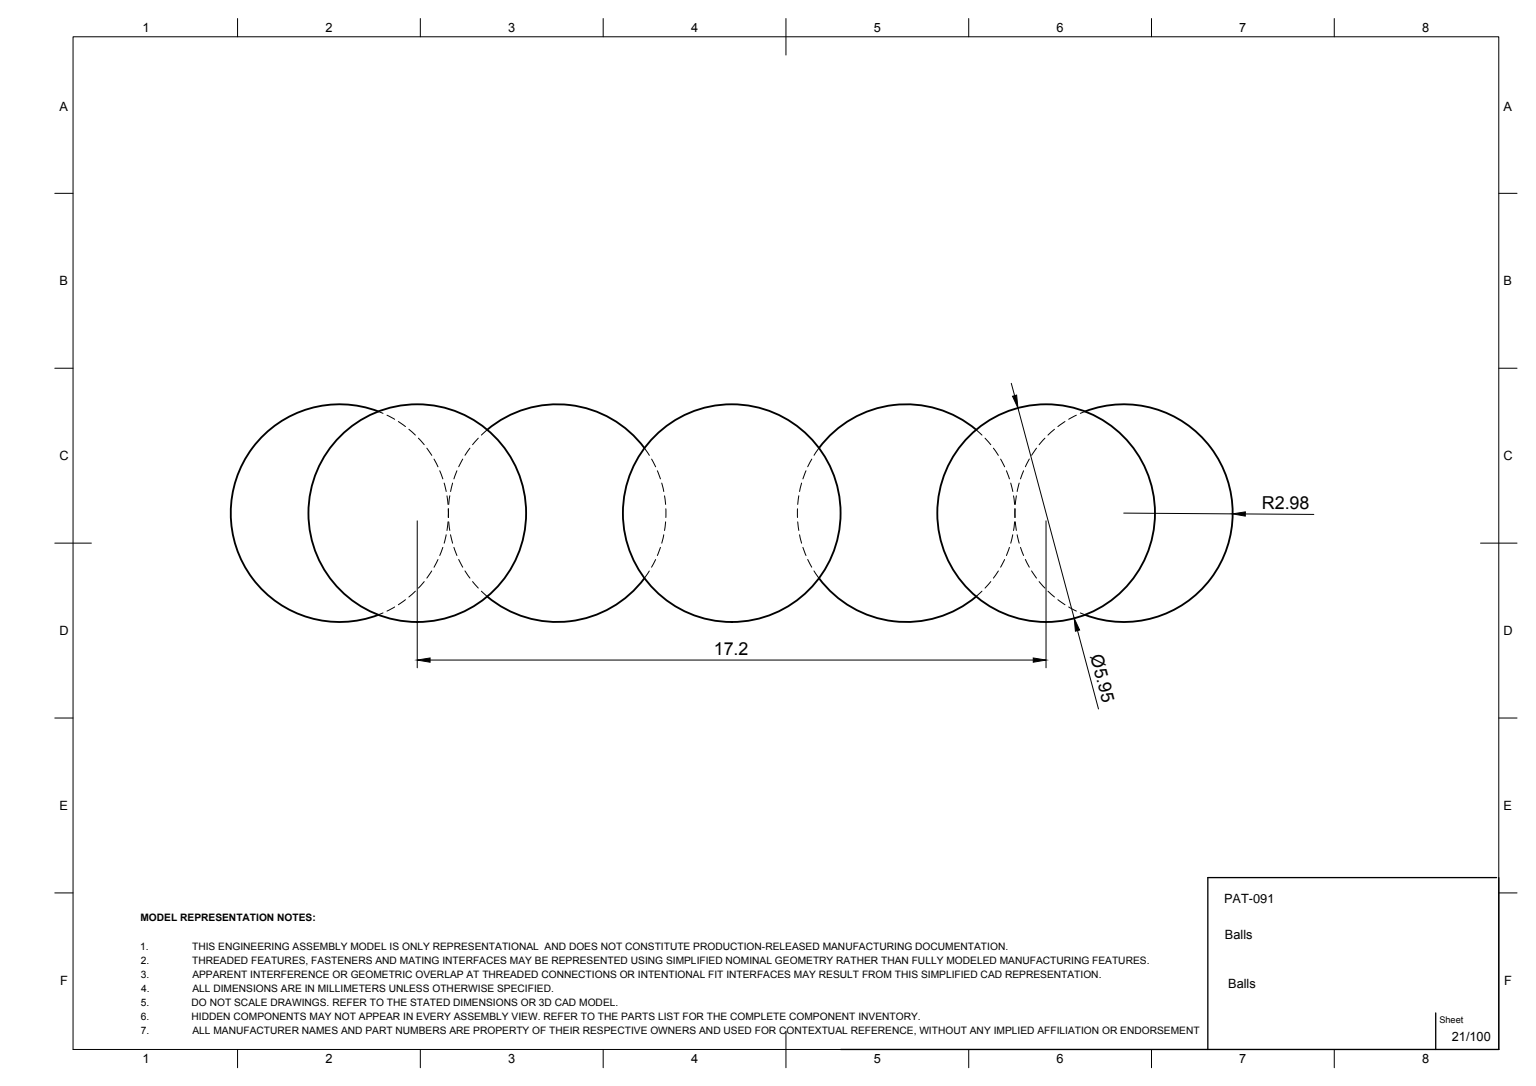
ISO-10303-21;
HEADER;
/* Generated by software containing ST-Developer
 * from STEP Tools, Inc. (www.steptools.com) 
 */

FILE_DESCRIPTION(
/* description */ ('PAT-091'),
/* implementation_level */ '2;1');

FILE_NAME(
/* name */ 'Balls.step',
/* time_stamp */ '2026-10-27T15:34:44-07:00',
/* author */ (''),
/* organization */ (''),
/* preprocessor_version */ 'ST-DEVELOPER v20.2',
/* originating_system */ 'Autodesk Translation Framework v15.17.0.0',
/* authorisation */ '');

FILE_SCHEMA (('AUTOMOTIVE_DESIGN { 1 0 10303 214 3 1 1 }'));
ENDSEC;

DATA;
#10=MECHANICAL_DESIGN_GEOMETRIC_PRESENTATION_REPRESENTATION('',(#1072,#1073,#1074,#1075,#1076,#1077,#1078),#25100);
#14=SPHERICAL_SURFACE('',#16174,0.29765);
#15=SPHERICAL_SURFACE('',#16176,0.29765);
#16=SPHERICAL_SURFACE('',#16178,0.29765);
#17=SPHERICAL_SURFACE('',#16180,0.29765);
#18=SPHERICAL_SURFACE('',#16182,0.29765);
#19=SPHERICAL_SURFACE('',#16184,0.29765);
#20=SPHERICAL_SURFACE('',#16186,0.29765);
#852=SHAPE_REPRESENTATION_RELATIONSHIP('SRR','None',#25620,#962);
#962=ADVANCED_BREP_SHAPE_REPRESENTATION('',(#1193,#1194,#1195,#1196,#1197,
#1198,#1199),#25090);
#1072=STYLED_ITEM('',(#26191),#1193);
#1073=STYLED_ITEM('',(#26191),#1194);
#1074=STYLED_ITEM('',(#26191),#1195);
#1075=STYLED_ITEM('',(#26191),#1196);
#1076=STYLED_ITEM('',(#26191),#1197);
#1077=STYLED_ITEM('',(#26191),#1198);
#1078=STYLED_ITEM('',(#26191),#1199);
#1193=MANIFOLD_SOLID_BREP('Body1',#13352);
#1194=MANIFOLD_SOLID_BREP('Body2',#13353);
#1195=MANIFOLD_SOLID_BREP('Body3',#13354);
#1196=MANIFOLD_SOLID_BREP('Body4',#13355);
#1197=MANIFOLD_SOLID_BREP('Body5',#13356);
#1198=MANIFOLD_SOLID_BREP('Body6',#13357);
#1199=MANIFOLD_SOLID_BREP('Body7',#13358);
#2791=FACE_OUTER_BOUND('',#4015,.T.);
#2792=FACE_OUTER_BOUND('',#4016,.T.);
#2793=FACE_OUTER_BOUND('',#4017,.T.);
#2794=FACE_OUTER_BOUND('',#4018,.T.);
#2795=FACE_OUTER_BOUND('',#4019,.T.);
#2796=FACE_OUTER_BOUND('',#4020,.T.);
#2797=FACE_OUTER_BOUND('',#4021,.T.);
#4015=EDGE_LOOP('',(#11772,#11773));
#4016=EDGE_LOOP('',(#11774,#11775));
#4017=EDGE_LOOP('',(#11776,#11777));
#4018=EDGE_LOOP('',(#11778,#11779));
#4019=EDGE_LOOP('',(#11780,#11781));
#4020=EDGE_LOOP('',(#11782,#11783));
#4021=EDGE_LOOP('',(#11784,#11785));
#6280=CIRCLE('',#16175,0.29765);
#6281=CIRCLE('',#16177,0.29765);
#6282=CIRCLE('',#16179,0.29765);
#6283=CIRCLE('',#16181,0.29765);
#6284=CIRCLE('',#16183,0.29765);
#6285=CIRCLE('',#16185,0.29765);
#6286=CIRCLE('',#16187,0.29765);
#7311=VERTEX_POINT('',#24268);
#7312=VERTEX_POINT('',#24269);
#7313=VERTEX_POINT('',#24272);
#7314=VERTEX_POINT('',#24273);
#7315=VERTEX_POINT('',#24276);
#7316=VERTEX_POINT('',#24277);
#7317=VERTEX_POINT('',#24280);
#7318=VERTEX_POINT('',#24281);
#7319=VERTEX_POINT('',#24284);
#7320=VERTEX_POINT('',#24285);
#7321=VERTEX_POINT('',#24288);
#7322=VERTEX_POINT('',#24289);
#7323=VERTEX_POINT('',#24292);
#7324=VERTEX_POINT('',#24293);
#8821=EDGE_CURVE('',#7311,#7312,#6280,.T.);
#8822=EDGE_CURVE('',#7313,#7314,#6281,.T.);
#8823=EDGE_CURVE('',#7315,#7316,#6282,.T.);
#8824=EDGE_CURVE('',#7317,#7318,#6283,.T.);
#8825=EDGE_CURVE('',#7319,#7320,#6284,.T.);
#8826=EDGE_CURVE('',#7321,#7322,#6285,.T.);
#8827=EDGE_CURVE('',#7323,#7324,#6286,.T.);
#11772=ORIENTED_EDGE('',*,*,#8821,.T.);
#11773=ORIENTED_EDGE('',*,*,#8821,.F.);
#11774=ORIENTED_EDGE('',*,*,#8822,.T.);
#11775=ORIENTED_EDGE('',*,*,#8822,.F.);
#11776=ORIENTED_EDGE('',*,*,#8823,.T.);
#11777=ORIENTED_EDGE('',*,*,#8823,.F.);
#11778=ORIENTED_EDGE('',*,*,#8824,.T.);
#11779=ORIENTED_EDGE('',*,*,#8824,.F.);
#11780=ORIENTED_EDGE('',*,*,#8825,.T.);
#11781=ORIENTED_EDGE('',*,*,#8825,.F.);
#11782=ORIENTED_EDGE('',*,*,#8826,.T.);
#11783=ORIENTED_EDGE('',*,*,#8826,.F.);
#11784=ORIENTED_EDGE('',*,*,#8827,.T.);
#11785=ORIENTED_EDGE('',*,*,#8827,.F.);
#13158=ADVANCED_FACE('',(#2791),#14,.T.);
#13159=ADVANCED_FACE('',(#2792),#15,.T.);
#13160=ADVANCED_FACE('',(#2793),#16,.T.);
#13161=ADVANCED_FACE('',(#2794),#17,.T.);
#13162=ADVANCED_FACE('',(#2795),#18,.T.);
#13163=ADVANCED_FACE('',(#2796),#19,.T.);
#13164=ADVANCED_FACE('',(#2797),#20,.T.);
#13352=CLOSED_SHELL('',(#13158));
#13353=CLOSED_SHELL('',(#13159));
#13354=CLOSED_SHELL('',(#13160));
#13355=CLOSED_SHELL('',(#13161));
#13356=CLOSED_SHELL('',(#13162));
#13357=CLOSED_SHELL('',(#13163));
#13358=CLOSED_SHELL('',(#13164));
#16173=AXIS2_PLACEMENT_3D('',#24266,#20364,#20365);
#16174=AXIS2_PLACEMENT_3D('',#24267,#20366,#20367);
#16175=AXIS2_PLACEMENT_3D('',#24270,#20368,#20369);
#16176=AXIS2_PLACEMENT_3D('',#24271,#20370,#20371);
#16177=AXIS2_PLACEMENT_3D('',#24274,#20372,#20373);
#16178=AXIS2_PLACEMENT_3D('',#24275,#20374,#20375);
#16179=AXIS2_PLACEMENT_3D('',#24278,#20376,#20377);
#16180=AXIS2_PLACEMENT_3D('',#24279,#20378,#20379);
#16181=AXIS2_PLACEMENT_3D('',#24282,#20380,#20381);
#16182=AXIS2_PLACEMENT_3D('',#24283,#20382,#20383);
#16183=AXIS2_PLACEMENT_3D('',#24286,#20384,#20385);
#16184=AXIS2_PLACEMENT_3D('',#24287,#20386,#20387);
#16185=AXIS2_PLACEMENT_3D('',#24290,#20388,#20389);
#16186=AXIS2_PLACEMENT_3D('',#24291,#20390,#20391);
#16187=AXIS2_PLACEMENT_3D('',#24294,#20392,#20393);
#20364=DIRECTION('axis',(0.,0.,1.));
#20365=DIRECTION('refdir',(1.,0.,0.));
#20366=DIRECTION('center_axis',(0.,0.,1.));
#20367=DIRECTION('ref_axis',(1.,0.,0.));
#20368=DIRECTION('center_axis',(1.22464679914735E-16,-1.,0.));
#20369=DIRECTION('ref_axis',(-1.,-1.22464679914735E-16,0.));
#20370=DIRECTION('center_axis',(0.78183148246803,0.,0.623489801858733));
#20371=DIRECTION('ref_axis',(0.623489801858734,0.,-0.78183148246803));
#20372=DIRECTION('center_axis',(7.63554790147315E-17,-1.,-9.57467422477103E-17));
#20373=DIRECTION('ref_axis',(-0.623489801858734,-1.22464679914735E-16,0.78183148246803));
#20374=DIRECTION('center_axis',(0.974927912181824,0.,-0.222520933956314));
#20375=DIRECTION('ref_axis',(-0.222520933956314,0.,-0.974927912181824));
#20376=DIRECTION('center_axis',(-2.7250954951288E-17,-1.,-1.19394234705288E-16));
#20377=DIRECTION('ref_axis',(0.222520933956314,-1.22464679914735E-16,0.974927912181824));
#20378=DIRECTION('center_axis',(0.433883739117558,0.,-0.900968867902419));
#20379=DIRECTION('ref_axis',(-0.900968867902419,0.,-0.433883739117558));
#20380=DIRECTION('center_axis',(-1.10336864020811E-16,-1.,-5.31354332312403E-17));
#20381=DIRECTION('ref_axis',(0.900968867902419,-1.22464679914735E-16,0.433883739117558));
#20382=DIRECTION('center_axis',(-0.433883739117558,0.,-0.900968867902419));
#20383=DIRECTION('ref_axis',(-0.900968867902419,0.,0.433883739117558));
#20384=DIRECTION('center_axis',(-1.10336864020811E-16,-1.,5.31354332312403E-17));
#20385=DIRECTION('ref_axis',(0.900968867902419,-1.22464679914735E-16,-0.433883739117558));
#20386=DIRECTION('center_axis',(-0.974927912181824,0.,-0.222520933956314));
#20387=DIRECTION('ref_axis',(-0.222520933956315,0.,0.974927912181824));
#20388=DIRECTION('center_axis',(-2.7250954951288E-17,-1.,1.19394234705288E-16));
#20389=DIRECTION('ref_axis',(0.222520933956315,-1.22464679914735E-16,-0.974927912181824));
#20390=DIRECTION('center_axis',(-0.78183148246803,0.,0.623489801858734));
#20391=DIRECTION('ref_axis',(0.623489801858733,0.,0.78183148246803));
#20392=DIRECTION('center_axis',(7.63554790147315E-17,-1.,9.57467422477103E-17));
#20393=DIRECTION('ref_axis',(-0.623489801858733,-1.22464679914735E-16,-0.78183148246803));
#24266=CARTESIAN_POINT('',(0.,0.,0.));
#24267=CARTESIAN_POINT('Origin',(1.1,0.,0.));
#24268=CARTESIAN_POINT('',(1.1,-2.23201749654651E-33,0.29765));
#24269=CARTESIAN_POINT('',(1.1,-2.23201749654651E-33,-0.29765));
#24270=CARTESIAN_POINT('Origin',(1.1,0.,0.));
#24271=CARTESIAN_POINT('Origin',(0.685838782044607,0.,-0.860014630714833));
#24272=CARTESIAN_POINT('',(0.918550922801216,-5.31350540756609E-33,-0.674432891191581));
#24273=CARTESIAN_POINT('',(0.453126641287998,8.49470414473068E-34,-1.04559637023808));
#24274=CARTESIAN_POINT('Origin',(0.685838782044607,0.,-0.860014630714833));
#24275=CARTESIAN_POINT('Origin',(-0.244773027351946,0.,-1.07242070340001));
#24276=CARTESIAN_POINT('',(0.0454142657089739,-2.23201749654651E-33,-1.1386540593921));
#24277=CARTESIAN_POINT('',(-0.534960320412865,-2.23201749654651E-33,-1.00618734740791));
#24278=CARTESIAN_POINT('Origin',(-0.244773027351946,0.,-1.07242070340001));
#24279=CARTESIAN_POINT('Origin',(-0.991065754692661,0.,-0.477272113029314));
#24280=CARTESIAN_POINT('',(-0.86192025974432,8.49470414473067E-34,-0.745445496560469));
#24281=CARTESIAN_POINT('',(-1.120211249641,-5.31350540756609E-33,-0.209098729498159));
#24282=CARTESIAN_POINT('Origin',(-0.991065754692661,0.,-0.477272113029314));
#24283=CARTESIAN_POINT('Origin',(-0.991065754692661,0.,0.477272113029314));
#24284=CARTESIAN_POINT('',(-1.120211249641,-2.23201749654651E-33,0.209098729498159));
#24285=CARTESIAN_POINT('',(-0.86192025974432,-2.23201749654651E-33,0.745445496560469));
#24286=CARTESIAN_POINT('Origin',(-0.991065754692661,0.,0.477272113029314));
#24287=CARTESIAN_POINT('Origin',(-0.244773027351946,0.,1.07242070340001));
#24288=CARTESIAN_POINT('',(-0.534960320412866,-2.23201749654651E-33,1.00618734740791));
#24289=CARTESIAN_POINT('',(0.0454142657089737,-2.23201749654651E-33,1.1386540593921));
#24290=CARTESIAN_POINT('Origin',(-0.244773027351946,0.,1.07242070340001));
#24291=CARTESIAN_POINT('Origin',(0.685838782044607,0.,0.860014630714833));
#24292=CARTESIAN_POINT('',(0.453126641287998,-2.23201749654651E-33,1.04559637023808));
#24293=CARTESIAN_POINT('',(0.918550922801216,-2.23201749654651E-33,0.674432891191581));
#24294=CARTESIAN_POINT('Origin',(0.685838782044607,0.,0.860014630714833));
#24969=UNCERTAINTY_MEASURE_WITH_UNIT(LENGTH_MEASURE(0.001),#25101,
'DISTANCE_ACCURACY_VALUE',
'Maximum model space distance between geometric entities at asserted c
onnectivities');
#24979=UNCERTAINTY_MEASURE_WITH_UNIT(LENGTH_MEASURE(0.001),#25101,
'DISTANCE_ACCURACY_VALUE',
'Maximum model space distance between geometric entities at asserted c
onnectivities');
#25090=(
GEOMETRIC_REPRESENTATION_CONTEXT(3)
GLOBAL_UNCERTAINTY_ASSIGNED_CONTEXT((#24969))
GLOBAL_UNIT_ASSIGNED_CONTEXT((#25101,#25103,#25104))
REPRESENTATION_CONTEXT('','3D')
);
#25100=(
GEOMETRIC_REPRESENTATION_CONTEXT(3)
GLOBAL_UNCERTAINTY_ASSIGNED_CONTEXT((#24979))
GLOBAL_UNIT_ASSIGNED_CONTEXT((#25101,#25103,#25104))
REPRESENTATION_CONTEXT('','3D')
);
#25101=(
LENGTH_UNIT()
NAMED_UNIT(*)
SI_UNIT(.CENTI.,.METRE.)
);
#25103=(
NAMED_UNIT(*)
PLANE_ANGLE_UNIT()
SI_UNIT($,.RADIAN.)
);
#25104=(
NAMED_UNIT(*)
SI_UNIT($,.STERADIAN.)
SOLID_ANGLE_UNIT()
);
#25215=SHAPE_DEFINITION_REPRESENTATION(#25409,#25620);
#25409=PRODUCT_DEFINITION_SHAPE('',$,#25741);
#25620=SHAPE_REPRESENTATION('',(#16173),#25090);
#25630=PRODUCT_DEFINITION_CONTEXT('part definition',#25992,'design');
#25741=PRODUCT_DEFINITION('Balls','Balls',#25861,#25630);
#25861=PRODUCT_DEFINITION_FORMATION('',$,#26104);
#25992=APPLICATION_CONTEXT(
'Core Data for Automotive Mechanical Design Process');
#25993=PRODUCT_CONTEXT('part definition',#25992,'mechanical');
#26104=PRODUCT('Balls','Balls','Balls',(#25993));
#26185=COLOUR_RGB('Grey',0.48,0.52,0.57);
#26186=FILL_AREA_STYLE_COLOUR('',#26185);
#26187=FILL_AREA_STYLE('',(#26186));
#26188=SURFACE_STYLE_FILL_AREA(#26187);
#26189=SURFACE_SIDE_STYLE('',(#26188));
#26190=SURFACE_STYLE_USAGE(.BOTH.,#26189);
#26191=PRESENTATION_STYLE_ASSIGNMENT((#26190));
ENDSEC;
END-ISO-10303-21;
